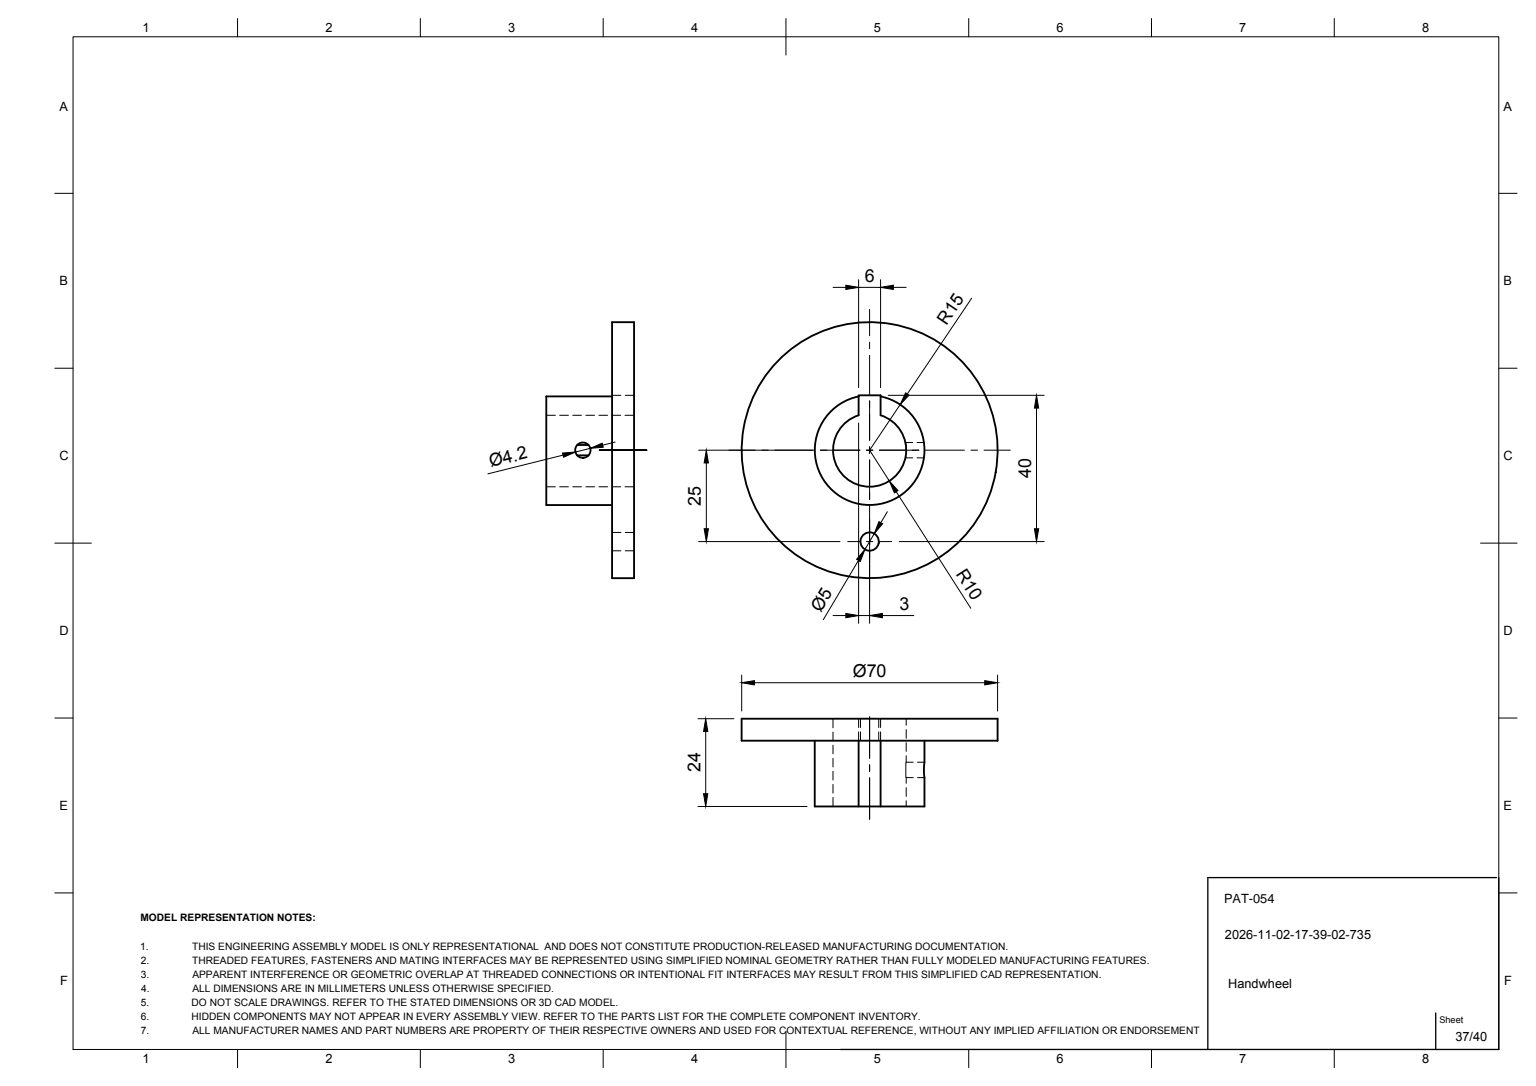
ISO-10303-21;
HEADER;
/* Generated by software containing ST-Developer
 * from STEP Tools, Inc. (www.steptools.com) 
 */

FILE_DESCRIPTION(
/* description */ ('PAT-054'),
/* implementation_level */ '2;1');

FILE_NAME(
/* name */ 'Handwheel.step',
/* time_stamp */ '2026-10-29T16:38:13-07:00',
/* author */ (''),
/* organization */ (''),
/* preprocessor_version */ 'ST-DEVELOPER v20.2',
/* originating_system */ 'Autodesk Translation Framework v15.17.0.0',
/* authorisation */ '');

FILE_SCHEMA (('AUTOMOTIVE_DESIGN { 1 0 10303 214 3 1 1 }'));
ENDSEC;

DATA;
#10=MECHANICAL_DESIGN_GEOMETRIC_PRESENTATION_REPRESENTATION('',(#951),#33981);
#742=B_SPLINE_CURVE_WITH_KNOTS('',3,(#33488,#33489,#33490,#33491,#33492,
#33493),.UNSPECIFIED.,.F.,.F.,(4,2,4),(0.803821788694078,0.872950991853625,
0.952307212900975),.UNSPECIFIED.);
#743=B_SPLINE_CURVE_WITH_KNOTS('',3,(#33496,#33497,#33498,#33499,#33500,
#33501,#33502,#33503,#33504,#33505),.UNSPECIFIED.,.F.,.F.,(4,2,2,2,4),(0.168950313426762,
0.238079516586309,0.317435737633658,0.396791958681008,0.465921161840561),
 .UNSPECIFIED.);
#744=B_SPLINE_CURVE_WITH_KNOTS('',3,(#33506,#33507,#33508,#33509,#33510,
#33511),.UNSPECIFIED.,.F.,.F.,(4,2,4),(0.952307212900975,1.03166343394832,
1.10079263710787),.UNSPECIFIED.);
#745=B_SPLINE_CURVE_WITH_KNOTS('',3,(#33515,#33516,#33517,#33518,#33519,
#33520,#33521,#33522,#33523,#33524),.UNSPECIFIED.,.F.,.F.,(4,2,2,2,4),(0.,
0.0792165807733642,0.158433161546728,0.237648697074572,0.316864232602417),
 .UNSPECIFIED.);
#746=B_SPLINE_CURVE_WITH_KNOTS('',3,(#33525,#33526,#33527,#33528,#33529,
#33530,#33531,#33532,#33533,#33534,#33535,#33536,#33537,#33538,#33539,#33540,
#33541,#33542,#33543,#33544,#33545,#33546,#33547,#33548,#33549,#33550),
 .UNSPECIFIED.,.F.,.F.,(4,2,2,2,2,2,2,2,2,2,2,2,4),(0.316864232602417,0.396079768130261,
0.475295303658105,0.554511884431469,0.633728465204833,0.712945045978197,
0.792161626751562,0.871377162279406,0.95059269780725,1.02980823333509,1.10902376886294,
1.1882403496363,1.26745693040967),.UNSPECIFIED.);
#848=SHAPE_REPRESENTATION_RELATIONSHIP('SRR','None',#34226,#892);
#892=ADVANCED_BREP_SHAPE_REPRESENTATION('',(#1006),#33974);
#951=STYLED_ITEM('',(#34510),#1006);
#1006=MANIFOLD_SOLID_BREP('Body1',#13066);
#1214=FACE_BOUND('',#3167,.T.);
#1215=FACE_BOUND('',#3168,.T.);
#1216=FACE_BOUND('',#3170,.T.);
#1217=FACE_BOUND('',#3171,.T.);
#1218=FACE_BOUND('',#3174,.T.);
#1219=FACE_BOUND('',#3176,.T.);
#1531=PLANE('',#14728);
#1532=PLANE('',#14732);
#1533=PLANE('',#14733);
#1534=PLANE('',#14734);
#1535=PLANE('',#14735);
#1536=PLANE('',#14736);
#1537=PLANE('',#14739);
#1538=PLANE('',#14747);
#2234=FACE_OUTER_BOUND('',#3159,.T.);
#2235=FACE_OUTER_BOUND('',#3160,.T.);
#2236=FACE_OUTER_BOUND('',#3161,.T.);
#2237=FACE_OUTER_BOUND('',#3162,.T.);
#2238=FACE_OUTER_BOUND('',#3163,.T.);
#2239=FACE_OUTER_BOUND('',#3164,.T.);
#2240=FACE_OUTER_BOUND('',#3165,.T.);
#2241=FACE_OUTER_BOUND('',#3166,.T.);
#2242=FACE_OUTER_BOUND('',#3169,.T.);
#2243=FACE_OUTER_BOUND('',#3172,.T.);
#2244=FACE_OUTER_BOUND('',#3173,.T.);
#2245=FACE_OUTER_BOUND('',#3175,.T.);
#2246=FACE_OUTER_BOUND('',#3177,.T.);
#3159=EDGE_LOOP('',(#11713,#11714,#11715,#11716));
#3160=EDGE_LOOP('',(#11717,#11718));
#3161=EDGE_LOOP('',(#11719,#11720,#11721,#11722,#11723,#11724,#11725,#11726,
#11727));
#3162=EDGE_LOOP('',(#11728,#11729));
#3163=EDGE_LOOP('',(#11730,#11731,#11732,#11733,#11734,#11735));
#3164=EDGE_LOOP('',(#11736,#11737,#11738,#11739));
#3165=EDGE_LOOP('',(#11740,#11741,#11742,#11743,#11744,#11745));
#3166=EDGE_LOOP('',(#11746));
#3167=EDGE_LOOP('',(#11747));
#3168=EDGE_LOOP('',(#11748,#11749,#11750,#11751));
#3169=EDGE_LOOP('',(#11752));
#3170=EDGE_LOOP('',(#11753));
#3171=EDGE_LOOP('',(#11754,#11755,#11756,#11757));
#3172=EDGE_LOOP('',(#11758,#11759,#11760,#11761));
#3173=EDGE_LOOP('',(#11762,#11763,#11764,#11765));
#3174=EDGE_LOOP('',(#11766,#11767,#11768,#11769,#11770));
#3175=EDGE_LOOP('',(#11771,#11772,#11773,#11774));
#3176=EDGE_LOOP('',(#11775,#11776));
#3177=EDGE_LOOP('',(#11777,#11778,#11779,#11780));
#4077=LINE('',#33478,#5011);
#4078=LINE('',#33483,#5012);
#4079=LINE('',#33513,#5013);
#4080=LINE('',#33552,#5014);
#4081=LINE('',#33556,#5015);
#4082=LINE('',#33558,#5016);
#4083=LINE('',#33560,#5017);
#4084=LINE('',#33562,#5018);
#4085=LINE('',#33564,#5019);
#4086=LINE('',#33565,#5020);
#4087=LINE('',#33568,#5021);
#4088=LINE('',#33570,#5022);
#4089=LINE('',#33571,#5023);
#4090=LINE('',#33574,#5024);
#4091=LINE('',#33576,#5025);
#4092=LINE('',#33578,#5026);
#4093=LINE('',#33580,#5027);
#4094=LINE('',#33581,#5028);
#4095=LINE('',#33591,#5029);
#5011=VECTOR('',#18066,0.25);
#5012=VECTOR('',#18071,1.);
#5013=VECTOR('',#18078,0.210000000000001);
#5014=VECTOR('',#18081,1.);
#5015=VECTOR('',#18084,1.);
#5016=VECTOR('',#18085,1.);
#5017=VECTOR('',#18086,1.);
#5018=VECTOR('',#18087,1.);
#5019=VECTOR('',#18088,1.);
#5020=VECTOR('',#18089,1.);
#5021=VECTOR('',#18092,1.);
#5022=VECTOR('',#18093,1.);
#5023=VECTOR('',#18094,1.);
#5024=VECTOR('',#18097,1.);
#5025=VECTOR('',#18098,1.);
#5026=VECTOR('',#18099,1.);
#5027=VECTOR('',#18100,1.);
#5028=VECTOR('',#18101,1.);
#5029=VECTOR('',#18116,3.5);
#5536=CIRCLE('',#14726,0.25);
#5537=CIRCLE('',#14727,0.25);
#5538=CIRCLE('',#14729,0.210000000000001);
#5539=CIRCLE('',#14731,0.210000000000001);
#5540=CIRCLE('',#14737,3.5);
#5541=CIRCLE('',#14738,1.);
#5542=CIRCLE('',#14740,3.5);
#5543=CIRCLE('',#14741,1.5);
#5544=CIRCLE('',#14744,1.);
#5545=CIRCLE('',#14746,1.5);
#6657=VERTEX_POINT('',#33475);
#6658=VERTEX_POINT('',#33477);
#6659=VERTEX_POINT('',#33481);
#6660=VERTEX_POINT('',#33482);
#6661=VERTEX_POINT('',#33486);
#6662=VERTEX_POINT('',#33487);
#6663=VERTEX_POINT('',#33494);
#6664=VERTEX_POINT('',#33512);
#6665=VERTEX_POINT('',#33514);
#6666=VERTEX_POINT('',#33554);
#6667=VERTEX_POINT('',#33555);
#6668=VERTEX_POINT('',#33557);
#6669=VERTEX_POINT('',#33559);
#6670=VERTEX_POINT('',#33561);
#6671=VERTEX_POINT('',#33563);
#6672=VERTEX_POINT('',#33567);
#6673=VERTEX_POINT('',#33569);
#6674=VERTEX_POINT('',#33573);
#6675=VERTEX_POINT('',#33575);
#6676=VERTEX_POINT('',#33577);
#6677=VERTEX_POINT('',#33579);
#6678=VERTEX_POINT('',#33583);
#6679=VERTEX_POINT('',#33587);
#8356=EDGE_CURVE('',#6657,#6657,#5536,.T.);
#8357=EDGE_CURVE('',#6657,#6658,#4077,.T.);
#8358=EDGE_CURVE('',#6658,#6658,#5537,.T.);
#8359=EDGE_CURVE('',#6659,#6660,#4078,.T.);
#8360=EDGE_CURVE('',#6659,#6660,#5538,.T.);
#8361=EDGE_CURVE('',#6661,#6662,#742,.T.);
#8362=EDGE_CURVE('',#6663,#6661,#5539,.T.);
#8363=EDGE_CURVE('',#6660,#6663,#743,.T.);
#8364=EDGE_CURVE('',#6662,#6659,#744,.T.);
#8365=EDGE_CURVE('',#6662,#6664,#4079,.T.);
#8366=EDGE_CURVE('',#6665,#6664,#745,.T.);
#8367=EDGE_CURVE('',#6664,#6665,#746,.T.);
#8368=EDGE_CURVE('',#6663,#6661,#4080,.T.);
#8369=EDGE_CURVE('',#6666,#6667,#4081,.T.);
#8370=EDGE_CURVE('',#6668,#6666,#4082,.T.);
#8371=EDGE_CURVE('',#6669,#6668,#4083,.T.);
#8372=EDGE_CURVE('',#6670,#6669,#4084,.T.);
#8373=EDGE_CURVE('',#6671,#6670,#4085,.T.);
#8374=EDGE_CURVE('',#6667,#6671,#4086,.T.);
#8375=EDGE_CURVE('',#6672,#6666,#4087,.T.);
#8376=EDGE_CURVE('',#6673,#6672,#4088,.T.);
#8377=EDGE_CURVE('',#6668,#6673,#4089,.T.);
#8378=EDGE_CURVE('',#6674,#6672,#4090,.T.);
#8379=EDGE_CURVE('',#6675,#6674,#4091,.T.);
#8380=EDGE_CURVE('',#6676,#6675,#4092,.T.);
#8381=EDGE_CURVE('',#6677,#6676,#4093,.T.);
#8382=EDGE_CURVE('',#6673,#6677,#4094,.T.);
#8383=EDGE_CURVE('',#6678,#6678,#5540,.T.);
#8384=EDGE_CURVE('',#6667,#6674,#5541,.T.);
#8385=EDGE_CURVE('',#6679,#6679,#5542,.T.);
#8386=EDGE_CURVE('',#6677,#6669,#5543,.T.);
#8387=EDGE_CURVE('',#6678,#6679,#4095,.T.);
#8388=EDGE_CURVE('',#6671,#6675,#5544,.T.);
#8389=EDGE_CURVE('',#6676,#6670,#5545,.T.);
#11713=ORIENTED_EDGE('',*,*,#8356,.F.);
#11714=ORIENTED_EDGE('',*,*,#8357,.T.);
#11715=ORIENTED_EDGE('',*,*,#8358,.F.);
#11716=ORIENTED_EDGE('',*,*,#8357,.F.);
#11717=ORIENTED_EDGE('',*,*,#8359,.F.);
#11718=ORIENTED_EDGE('',*,*,#8360,.T.);
#11719=ORIENTED_EDGE('',*,*,#8361,.F.);
#11720=ORIENTED_EDGE('',*,*,#8362,.F.);
#11721=ORIENTED_EDGE('',*,*,#8363,.F.);
#11722=ORIENTED_EDGE('',*,*,#8360,.F.);
#11723=ORIENTED_EDGE('',*,*,#8364,.F.);
#11724=ORIENTED_EDGE('',*,*,#8365,.T.);
#11725=ORIENTED_EDGE('',*,*,#8366,.F.);
#11726=ORIENTED_EDGE('',*,*,#8367,.F.);
#11727=ORIENTED_EDGE('',*,*,#8365,.F.);
#11728=ORIENTED_EDGE('',*,*,#8368,.F.);
#11729=ORIENTED_EDGE('',*,*,#8362,.T.);
#11730=ORIENTED_EDGE('',*,*,#8369,.F.);
#11731=ORIENTED_EDGE('',*,*,#8370,.F.);
#11732=ORIENTED_EDGE('',*,*,#8371,.F.);
#11733=ORIENTED_EDGE('',*,*,#8372,.F.);
#11734=ORIENTED_EDGE('',*,*,#8373,.F.);
#11735=ORIENTED_EDGE('',*,*,#8374,.F.);
#11736=ORIENTED_EDGE('',*,*,#8375,.F.);
#11737=ORIENTED_EDGE('',*,*,#8376,.F.);
#11738=ORIENTED_EDGE('',*,*,#8377,.F.);
#11739=ORIENTED_EDGE('',*,*,#8370,.T.);
#11740=ORIENTED_EDGE('',*,*,#8378,.F.);
#11741=ORIENTED_EDGE('',*,*,#8379,.F.);
#11742=ORIENTED_EDGE('',*,*,#8380,.F.);
#11743=ORIENTED_EDGE('',*,*,#8381,.F.);
#11744=ORIENTED_EDGE('',*,*,#8382,.F.);
#11745=ORIENTED_EDGE('',*,*,#8376,.T.);
#11746=ORIENTED_EDGE('',*,*,#8383,.T.);
#11747=ORIENTED_EDGE('',*,*,#8358,.T.);
#11748=ORIENTED_EDGE('',*,*,#8378,.T.);
#11749=ORIENTED_EDGE('',*,*,#8375,.T.);
#11750=ORIENTED_EDGE('',*,*,#8369,.T.);
#11751=ORIENTED_EDGE('',*,*,#8384,.T.);
#11752=ORIENTED_EDGE('',*,*,#8385,.F.);
#11753=ORIENTED_EDGE('',*,*,#8356,.T.);
#11754=ORIENTED_EDGE('',*,*,#8382,.T.);
#11755=ORIENTED_EDGE('',*,*,#8386,.T.);
#11756=ORIENTED_EDGE('',*,*,#8371,.T.);
#11757=ORIENTED_EDGE('',*,*,#8377,.T.);
#11758=ORIENTED_EDGE('',*,*,#8383,.F.);
#11759=ORIENTED_EDGE('',*,*,#8387,.T.);
#11760=ORIENTED_EDGE('',*,*,#8385,.T.);
#11761=ORIENTED_EDGE('',*,*,#8387,.F.);
#11762=ORIENTED_EDGE('',*,*,#8379,.T.);
#11763=ORIENTED_EDGE('',*,*,#8384,.F.);
#11764=ORIENTED_EDGE('',*,*,#8374,.T.);
#11765=ORIENTED_EDGE('',*,*,#8388,.T.);
#11766=ORIENTED_EDGE('',*,*,#8363,.T.);
#11767=ORIENTED_EDGE('',*,*,#8368,.T.);
#11768=ORIENTED_EDGE('',*,*,#8361,.T.);
#11769=ORIENTED_EDGE('',*,*,#8364,.T.);
#11770=ORIENTED_EDGE('',*,*,#8359,.T.);
#11771=ORIENTED_EDGE('',*,*,#8381,.T.);
#11772=ORIENTED_EDGE('',*,*,#8389,.T.);
#11773=ORIENTED_EDGE('',*,*,#8372,.T.);
#11774=ORIENTED_EDGE('',*,*,#8386,.F.);
#11775=ORIENTED_EDGE('',*,*,#8366,.T.);
#11776=ORIENTED_EDGE('',*,*,#8367,.T.);
#11777=ORIENTED_EDGE('',*,*,#8380,.T.);
#11778=ORIENTED_EDGE('',*,*,#8388,.F.);
#11779=ORIENTED_EDGE('',*,*,#8373,.T.);
#11780=ORIENTED_EDGE('',*,*,#8389,.F.);
#12273=CYLINDRICAL_SURFACE('',#14725,0.25);
#12274=CYLINDRICAL_SURFACE('',#14730,0.210000000000001);
#12275=CYLINDRICAL_SURFACE('',#14742,3.5);
#12276=CYLINDRICAL_SURFACE('',#14743,1.);
#12277=CYLINDRICAL_SURFACE('',#14745,1.5);
#12946=ADVANCED_FACE('',(#2234),#12273,.F.);
#12947=ADVANCED_FACE('',(#2235),#1531,.T.);
#12948=ADVANCED_FACE('',(#2236),#12274,.F.);
#12949=ADVANCED_FACE('',(#2237),#1532,.T.);
#12950=ADVANCED_FACE('',(#2238),#1533,.F.);
#12951=ADVANCED_FACE('',(#2239),#1534,.F.);
#12952=ADVANCED_FACE('',(#2240),#1535,.F.);
#12953=ADVANCED_FACE('',(#2241,#1214,#1215),#1536,.T.);
#12954=ADVANCED_FACE('',(#2242,#1216,#1217),#1537,.F.);
#12955=ADVANCED_FACE('',(#2243),#12275,.T.);
#12956=ADVANCED_FACE('',(#2244,#1218),#12276,.F.);
#12957=ADVANCED_FACE('',(#2245,#1219),#12277,.T.);
#12958=ADVANCED_FACE('',(#2246),#1538,.F.);
#13066=CLOSED_SHELL('',(#12946,#12947,#12948,#12949,#12950,#12951,#12952,
#12953,#12954,#12955,#12956,#12957,#12958));
#14724=AXIS2_PLACEMENT_3D('',#33473,#18060,#18061);
#14725=AXIS2_PLACEMENT_3D('',#33474,#18062,#18063);
#14726=AXIS2_PLACEMENT_3D('',#33476,#18064,#18065);
#14727=AXIS2_PLACEMENT_3D('',#33479,#18067,#18068);
#14728=AXIS2_PLACEMENT_3D('',#33480,#18069,#18070);
#14729=AXIS2_PLACEMENT_3D('',#33484,#18072,#18073);
#14730=AXIS2_PLACEMENT_3D('',#33485,#18074,#18075);
#14731=AXIS2_PLACEMENT_3D('',#33495,#18076,#18077);
#14732=AXIS2_PLACEMENT_3D('',#33551,#18079,#18080);
#14733=AXIS2_PLACEMENT_3D('',#33553,#18082,#18083);
#14734=AXIS2_PLACEMENT_3D('',#33566,#18090,#18091);
#14735=AXIS2_PLACEMENT_3D('',#33572,#18095,#18096);
#14736=AXIS2_PLACEMENT_3D('',#33582,#18102,#18103);
#14737=AXIS2_PLACEMENT_3D('',#33584,#18104,#18105);
#14738=AXIS2_PLACEMENT_3D('',#33585,#18106,#18107);
#14739=AXIS2_PLACEMENT_3D('',#33586,#18108,#18109);
#14740=AXIS2_PLACEMENT_3D('',#33588,#18110,#18111);
#14741=AXIS2_PLACEMENT_3D('',#33589,#18112,#18113);
#14742=AXIS2_PLACEMENT_3D('',#33590,#18114,#18115);
#14743=AXIS2_PLACEMENT_3D('',#33592,#18117,#18118);
#14744=AXIS2_PLACEMENT_3D('',#33593,#18119,#18120);
#14745=AXIS2_PLACEMENT_3D('',#33594,#18121,#18122);
#14746=AXIS2_PLACEMENT_3D('',#33595,#18123,#18124);
#14747=AXIS2_PLACEMENT_3D('',#33596,#18125,#18126);
#18060=DIRECTION('axis',(0.,0.,1.));
#18061=DIRECTION('refdir',(1.,0.,0.));
#18062=DIRECTION('center_axis',(1.,0.,0.));
#18063=DIRECTION('ref_axis',(0.,0.,-1.));
#18064=DIRECTION('center_axis',(1.,0.,0.));
#18065=DIRECTION('ref_axis',(0.,0.,-1.));
#18066=DIRECTION('',(1.,0.,0.));
#18067=DIRECTION('center_axis',(-1.,0.,0.));
#18068=DIRECTION('ref_axis',(0.,0.,-1.));
#18069=DIRECTION('center_axis',(0.,1.,0.));
#18070=DIRECTION('ref_axis',(1.,0.,0.));
#18071=DIRECTION('',(1.,0.,0.));
#18072=DIRECTION('center_axis',(0.,1.,0.));
#18073=DIRECTION('ref_axis',(1.,0.,0.));
#18074=DIRECTION('center_axis',(0.,1.,0.));
#18075=DIRECTION('ref_axis',(1.,0.,0.));
#18076=DIRECTION('center_axis',(0.,1.,0.));
#18077=DIRECTION('ref_axis',(1.,0.,0.));
#18078=DIRECTION('',(0.,1.,0.));
#18079=DIRECTION('center_axis',(0.,1.,0.));
#18080=DIRECTION('ref_axis',(1.,0.,0.));
#18081=DIRECTION('',(-1.,0.,0.));
#18082=DIRECTION('center_axis',(0.,-1.,0.));
#18083=DIRECTION('ref_axis',(0.,0.,-1.));
#18084=DIRECTION('',(0.,0.,1.));
#18085=DIRECTION('',(1.,0.,0.));
#18086=DIRECTION('',(0.,0.,-1.));
#18087=DIRECTION('',(1.,0.,0.));
#18088=DIRECTION('',(0.,0.,-1.));
#18089=DIRECTION('',(-1.,0.,0.));
#18090=DIRECTION('center_axis',(0.,0.,-1.));
#18091=DIRECTION('ref_axis',(0.,1.,0.));
#18092=DIRECTION('',(0.,-1.,0.));
#18093=DIRECTION('',(1.,0.,0.));
#18094=DIRECTION('',(0.,1.,0.));
#18095=DIRECTION('center_axis',(0.,1.,0.));
#18096=DIRECTION('ref_axis',(0.,0.,1.));
#18097=DIRECTION('',(0.,0.,-1.));
#18098=DIRECTION('',(1.,0.,0.));
#18099=DIRECTION('',(0.,0.,1.));
#18100=DIRECTION('',(-1.,0.,0.));
#18101=DIRECTION('',(0.,0.,1.));
#18102=DIRECTION('center_axis',(1.,0.,0.));
#18103=DIRECTION('ref_axis',(0.,0.,-1.));
#18104=DIRECTION('center_axis',(1.,0.,0.));
#18105=DIRECTION('ref_axis',(0.,0.,-1.));
#18106=DIRECTION('center_axis',(-1.,0.,0.));
#18107=DIRECTION('ref_axis',(0.,0.,-1.));
#18108=DIRECTION('center_axis',(1.,0.,0.));
#18109=DIRECTION('ref_axis',(0.,0.,-1.));
#18110=DIRECTION('center_axis',(1.,0.,0.));
#18111=DIRECTION('ref_axis',(0.,0.,-1.));
#18112=DIRECTION('center_axis',(1.,0.,0.));
#18113=DIRECTION('ref_axis',(0.,0.,-1.));
#18114=DIRECTION('center_axis',(1.,0.,0.));
#18115=DIRECTION('ref_axis',(0.,0.,-1.));
#18116=DIRECTION('',(-1.,0.,0.));
#18117=DIRECTION('center_axis',(1.,0.,0.));
#18118=DIRECTION('ref_axis',(0.,1.22464679914735E-16,1.));
#18119=DIRECTION('center_axis',(-1.,0.,0.));
#18120=DIRECTION('ref_axis',(0.,0.,-1.));
#18121=DIRECTION('center_axis',(1.,0.,0.));
#18122=DIRECTION('ref_axis',(0.,1.22464679914735E-16,1.));
#18123=DIRECTION('center_axis',(1.,0.,0.));
#18124=DIRECTION('ref_axis',(0.,0.,-1.));
#18125=DIRECTION('center_axis',(1.,0.,0.));
#18126=DIRECTION('ref_axis',(0.,0.,-1.));
#33473=CARTESIAN_POINT('',(0.,0.,0.));
#33474=CARTESIAN_POINT('Origin',(28.7,0.,6.5));
#33475=CARTESIAN_POINT('',(28.8,-3.06161699786838E-17,6.75));
#33476=CARTESIAN_POINT('Origin',(28.8,0.,6.5));
#33477=CARTESIAN_POINT('',(29.4,3.06161699786838E-17,6.75));
#33478=CARTESIAN_POINT('',(28.7,-3.06161699786838E-17,6.75));
#33479=CARTESIAN_POINT('Origin',(29.4,0.,6.5));
#33480=CARTESIAN_POINT('Origin',(28.,0.99,4.));
#33481=CARTESIAN_POINT('',(27.844436508139,0.99,4.14106735979666));
#33482=CARTESIAN_POINT('',(28.155563491861,0.99,4.14106735979666));
#33483=CARTESIAN_POINT('',(27.,0.99,4.14106735979666));
#33484=CARTESIAN_POINT('Origin',(28.,0.99,4.));
#33485=CARTESIAN_POINT('Origin',(28.,0.99,4.));
#33486=CARTESIAN_POINT('',(27.844436508139,0.99,3.85893264020334));
#33487=CARTESIAN_POINT('',(27.79,1.,4.));
#33488=CARTESIAN_POINT('Ctrl Pts',(27.844436508139,0.99,3.85893264020334));
#33489=CARTESIAN_POINT('Ctrl Pts',(27.8287948476368,0.992457849824465,3.87618164330178));
#33490=CARTESIAN_POINT('Ctrl Pts',(27.815375956669,0.994938193049464,3.8970013568903));
#33491=CARTESIAN_POINT('Ctrl Pts',(27.7953025362756,0.998844492372413,3.94538588560165));
#33492=CARTESIAN_POINT('Ctrl Pts',(27.79,1.,3.97354792631755));
#33493=CARTESIAN_POINT('Ctrl Pts',(27.79,1.,4.));
#33494=CARTESIAN_POINT('',(28.155563491861,0.99,3.85893264020334));
#33495=CARTESIAN_POINT('Origin',(28.,0.99,4.));
#33496=CARTESIAN_POINT('Ctrl Pts',(28.155563491861,0.99,4.14106735979666));
#33497=CARTESIAN_POINT('Ctrl Pts',(28.1712051523632,0.992457849824465,4.12381835669823));
#33498=CARTESIAN_POINT('Ctrl Pts',(28.184624043331,0.994938193049464,4.1029986431097));
#33499=CARTESIAN_POINT('Ctrl Pts',(28.2046974637244,0.998844492372413,4.05461411439835));
#33500=CARTESIAN_POINT('Ctrl Pts',(28.21,1.,4.02645207368245));
#33501=CARTESIAN_POINT('Ctrl Pts',(28.21,1.,3.97354792631755));
#33502=CARTESIAN_POINT('Ctrl Pts',(28.2046974637244,0.998844492372413,3.94538588560165));
#33503=CARTESIAN_POINT('Ctrl Pts',(28.184624043331,0.994938193049464,3.8970013568903));
#33504=CARTESIAN_POINT('Ctrl Pts',(28.1712051523632,0.992457849824465,3.87618164330178));
#33505=CARTESIAN_POINT('Ctrl Pts',(28.155563491861,0.99,3.85893264020334));
#33506=CARTESIAN_POINT('Ctrl Pts',(27.79,1.,4.));
#33507=CARTESIAN_POINT('Ctrl Pts',(27.79,1.,4.02645207368245));
#33508=CARTESIAN_POINT('Ctrl Pts',(27.7953025362756,0.998844492372413,4.05461411439835));
#33509=CARTESIAN_POINT('Ctrl Pts',(27.815375956669,0.994938193049464,4.1029986431097));
#33510=CARTESIAN_POINT('Ctrl Pts',(27.8287948476368,0.992457849824465,4.12381835669823));
#33511=CARTESIAN_POINT('Ctrl Pts',(27.844436508139,0.99,4.14106735979666));
#33512=CARTESIAN_POINT('',(27.79,1.5,4.));
#33513=CARTESIAN_POINT('',(27.79,0.99,4.));
#33514=CARTESIAN_POINT('',(28.,1.48522725533839,4.21));
#33515=CARTESIAN_POINT('Ctrl Pts',(28.,1.48522725533839,4.21));
#33516=CARTESIAN_POINT('Ctrl Pts',(27.9735944730755,1.48522725533839,4.21));
#33517=CARTESIAN_POINT('Ctrl Pts',(27.9454529259093,1.48600415954412,4.20471573726959));
#33518=CARTESIAN_POINT('Ctrl Pts',(27.8937237310949,1.48880073282317,4.18327376303633));
#33519=CARTESIAN_POINT('Ctrl Pts',(27.870133075872,1.49077897157582,4.16711792397039));
#33520=CARTESIAN_POINT('Ctrl Pts',(27.832882321789,1.49448481141327,4.12986716988737));
#33521=CARTESIAN_POINT('Ctrl Pts',(27.8167262899986,1.49645455657129,4.10627640830576));
#33522=CARTESIAN_POINT('Ctrl Pts',(27.7952841751738,1.49923165515646,4.0545468514059));
#33523=CARTESIAN_POINT('Ctrl Pts',(27.79,1.5,4.02640517850928));
#33524=CARTESIAN_POINT('Ctrl Pts',(27.79,1.5,4.));
#33525=CARTESIAN_POINT('Ctrl Pts',(27.79,1.5,4.));
#33526=CARTESIAN_POINT('Ctrl Pts',(27.79,1.5,3.97359482149072));
#33527=CARTESIAN_POINT('Ctrl Pts',(27.7952841751738,1.49923165515646,3.9454531485941));
#33528=CARTESIAN_POINT('Ctrl Pts',(27.8167262899986,1.49645455657129,3.89372359169424));
#33529=CARTESIAN_POINT('Ctrl Pts',(27.832882321789,1.49448481141327,3.87013283011263));
#33530=CARTESIAN_POINT('Ctrl Pts',(27.870133075872,1.49077897157582,3.83288207602961));
#33531=CARTESIAN_POINT('Ctrl Pts',(27.8937237310949,1.48880073282317,3.81672623696367));
#33532=CARTESIAN_POINT('Ctrl Pts',(27.9454529259093,1.48600415954412,3.7952842627304));
#33533=CARTESIAN_POINT('Ctrl Pts',(27.9735944730755,1.48522725533839,3.79));
#33534=CARTESIAN_POINT('Ctrl Pts',(28.0264055269245,1.48522725533839,3.79));
#33535=CARTESIAN_POINT('Ctrl Pts',(28.0545470740907,1.48600415954412,3.7952842627304));
#33536=CARTESIAN_POINT('Ctrl Pts',(28.1062762689051,1.48880073282317,3.81672623696367));
#33537=CARTESIAN_POINT('Ctrl Pts',(28.129866924128,1.49077897157582,3.83288207602961));
#33538=CARTESIAN_POINT('Ctrl Pts',(28.167117678211,1.49448481141327,3.87013283011263));
#33539=CARTESIAN_POINT('Ctrl Pts',(28.1832737100014,1.49645455657129,3.89372359169424));
#33540=CARTESIAN_POINT('Ctrl Pts',(28.2047158248262,1.49923165515646,3.9454531485941));
#33541=CARTESIAN_POINT('Ctrl Pts',(28.21,1.5,3.97359482149072));
#33542=CARTESIAN_POINT('Ctrl Pts',(28.21,1.5,4.02640517850928));
#33543=CARTESIAN_POINT('Ctrl Pts',(28.2047158248262,1.49923165515646,4.0545468514059));
#33544=CARTESIAN_POINT('Ctrl Pts',(28.1832737100014,1.49645455657129,4.10627640830576));
#33545=CARTESIAN_POINT('Ctrl Pts',(28.167117678211,1.49448481141327,4.12986716988737));
#33546=CARTESIAN_POINT('Ctrl Pts',(28.129866924128,1.49077897157582,4.16711792397039));
#33547=CARTESIAN_POINT('Ctrl Pts',(28.1062762689051,1.48880073282317,4.18327376303633));
#33548=CARTESIAN_POINT('Ctrl Pts',(28.0545470740907,1.48600415954412,4.2047157372696));
#33549=CARTESIAN_POINT('Ctrl Pts',(28.0264055269245,1.48522725533839,4.21));
#33550=CARTESIAN_POINT('Ctrl Pts',(28.,1.48522725533839,4.21));
#33551=CARTESIAN_POINT('Origin',(28.,0.99,4.));
#33552=CARTESIAN_POINT('',(27.,0.99,3.85893264020334));
#33553=CARTESIAN_POINT('Origin',(26.9,-0.3,4.));
#33554=CARTESIAN_POINT('',(29.4,-0.3,2.5));
#33555=CARTESIAN_POINT('',(29.4,-0.3,3.04606079858305));
#33556=CARTESIAN_POINT('',(29.4,-0.3,4.));
#33557=CARTESIAN_POINT('',(28.8,-0.3,2.5));
#33558=CARTESIAN_POINT('',(26.9,-0.3,2.5));
#33559=CARTESIAN_POINT('',(28.8,-0.3,2.53030615433009));
#33560=CARTESIAN_POINT('',(28.8,-0.3,4.));
#33561=CARTESIAN_POINT('',(27.,-0.3,2.53030615433009));
#33562=CARTESIAN_POINT('',(27.,-0.3,2.53030615433009));
#33563=CARTESIAN_POINT('',(27.,-0.3,3.04606079858305));
#33564=CARTESIAN_POINT('',(27.,-0.3,4.));
#33565=CARTESIAN_POINT('',(27.,-0.3,3.04606079858305));
#33566=CARTESIAN_POINT('Origin',(26.9,-0.3,2.5));
#33567=CARTESIAN_POINT('',(29.4,0.3,2.5));
#33568=CARTESIAN_POINT('',(29.4,-0.15,2.5));
#33569=CARTESIAN_POINT('',(28.8,0.3,2.5));
#33570=CARTESIAN_POINT('',(26.9,0.3,2.5));
#33571=CARTESIAN_POINT('',(28.8,-0.15,2.5));
#33572=CARTESIAN_POINT('Origin',(26.9,0.3,2.5));
#33573=CARTESIAN_POINT('',(29.4,0.3,3.04606079858305));
#33574=CARTESIAN_POINT('',(29.4,0.3,3.25));
#33575=CARTESIAN_POINT('',(27.,0.3,3.04606079858305));
#33576=CARTESIAN_POINT('',(27.,0.3,3.04606079858305));
#33577=CARTESIAN_POINT('',(27.,0.3,2.53030615433009));
#33578=CARTESIAN_POINT('',(27.,0.3,3.25));
#33579=CARTESIAN_POINT('',(28.8,0.3,2.53030615433009));
#33580=CARTESIAN_POINT('',(27.,0.3,2.53030615433009));
#33581=CARTESIAN_POINT('',(28.8,0.3,3.25));
#33582=CARTESIAN_POINT('Origin',(29.4,0.,4.));
#33583=CARTESIAN_POINT('',(29.4,-4.28626379701574E-16,7.5));
#33584=CARTESIAN_POINT('Origin',(29.4,0.,4.));
#33585=CARTESIAN_POINT('Origin',(29.4,0.,4.));
#33586=CARTESIAN_POINT('Origin',(28.8,0.,4.));
#33587=CARTESIAN_POINT('',(28.8,-4.28626379701574E-16,7.5));
#33588=CARTESIAN_POINT('Origin',(28.8,0.,4.));
#33589=CARTESIAN_POINT('Origin',(28.8,0.,4.));
#33590=CARTESIAN_POINT('Origin',(28.8,0.,4.));
#33591=CARTESIAN_POINT('',(28.8,-4.28626379701574E-16,7.5));
#33592=CARTESIAN_POINT('Origin',(27.,0.,4.));
#33593=CARTESIAN_POINT('Origin',(27.,0.,4.));
#33594=CARTESIAN_POINT('Origin',(27.,0.,4.));
#33595=CARTESIAN_POINT('Origin',(27.,0.,4.));
#33596=CARTESIAN_POINT('Origin',(27.,0.,4.));
#33922=UNCERTAINTY_MEASURE_WITH_UNIT(LENGTH_MEASURE(0.001),#33982,
'DISTANCE_ACCURACY_VALUE',
'Maximum model space distance between geometric entities at asserted c
onnectivities');
#33929=UNCERTAINTY_MEASURE_WITH_UNIT(LENGTH_MEASURE(0.001),#33982,
'DISTANCE_ACCURACY_VALUE',
'Maximum model space distance between geometric entities at asserted c
onnectivities');
#33974=(
GEOMETRIC_REPRESENTATION_CONTEXT(3)
GLOBAL_UNCERTAINTY_ASSIGNED_CONTEXT((#33922))
GLOBAL_UNIT_ASSIGNED_CONTEXT((#33982,#33984,#33985))
REPRESENTATION_CONTEXT('','3D')
);
#33981=(
GEOMETRIC_REPRESENTATION_CONTEXT(3)
GLOBAL_UNCERTAINTY_ASSIGNED_CONTEXT((#33929))
GLOBAL_UNIT_ASSIGNED_CONTEXT((#33982,#33984,#33985))
REPRESENTATION_CONTEXT('','3D')
);
#33982=(
LENGTH_UNIT()
NAMED_UNIT(*)
SI_UNIT(.CENTI.,.METRE.)
);
#33984=(
NAMED_UNIT(*)
PLANE_ANGLE_UNIT()
SI_UNIT($,.RADIAN.)
);
#33985=(
NAMED_UNIT(*)
SI_UNIT($,.STERADIAN.)
SOLID_ANGLE_UNIT()
);
#34030=SHAPE_DEFINITION_REPRESENTATION(#34114,#34226);
#34114=PRODUCT_DEFINITION_SHAPE('',$,#34278);
#34226=SHAPE_REPRESENTATION('',(#14724),#33974);
#34233=PRODUCT_DEFINITION_CONTEXT('part definition',#34388,'design');
#34278=PRODUCT_DEFINITION('Handwheel','Handwheel',#34329,#34233);
#34329=PRODUCT_DEFINITION_FORMATION('',$,#34434);
#34388=APPLICATION_CONTEXT(
'Core Data for Automotive Mechanical Design Process');
#34389=PRODUCT_CONTEXT('part definition',#34388,'mechanical');
#34434=PRODUCT('Handwheel','Handwheel','Handwheel',(#34389));
#34504=COLOUR_RGB('Sky Blue',0.24,0.69,0.87);
#34505=FILL_AREA_STYLE_COLOUR('',#34504);
#34506=FILL_AREA_STYLE('',(#34505));
#34507=SURFACE_STYLE_FILL_AREA(#34506);
#34508=SURFACE_SIDE_STYLE('',(#34507));
#34509=SURFACE_STYLE_USAGE(.BOTH.,#34508);
#34510=PRESENTATION_STYLE_ASSIGNMENT((#34509));
ENDSEC;
END-ISO-10303-21;
